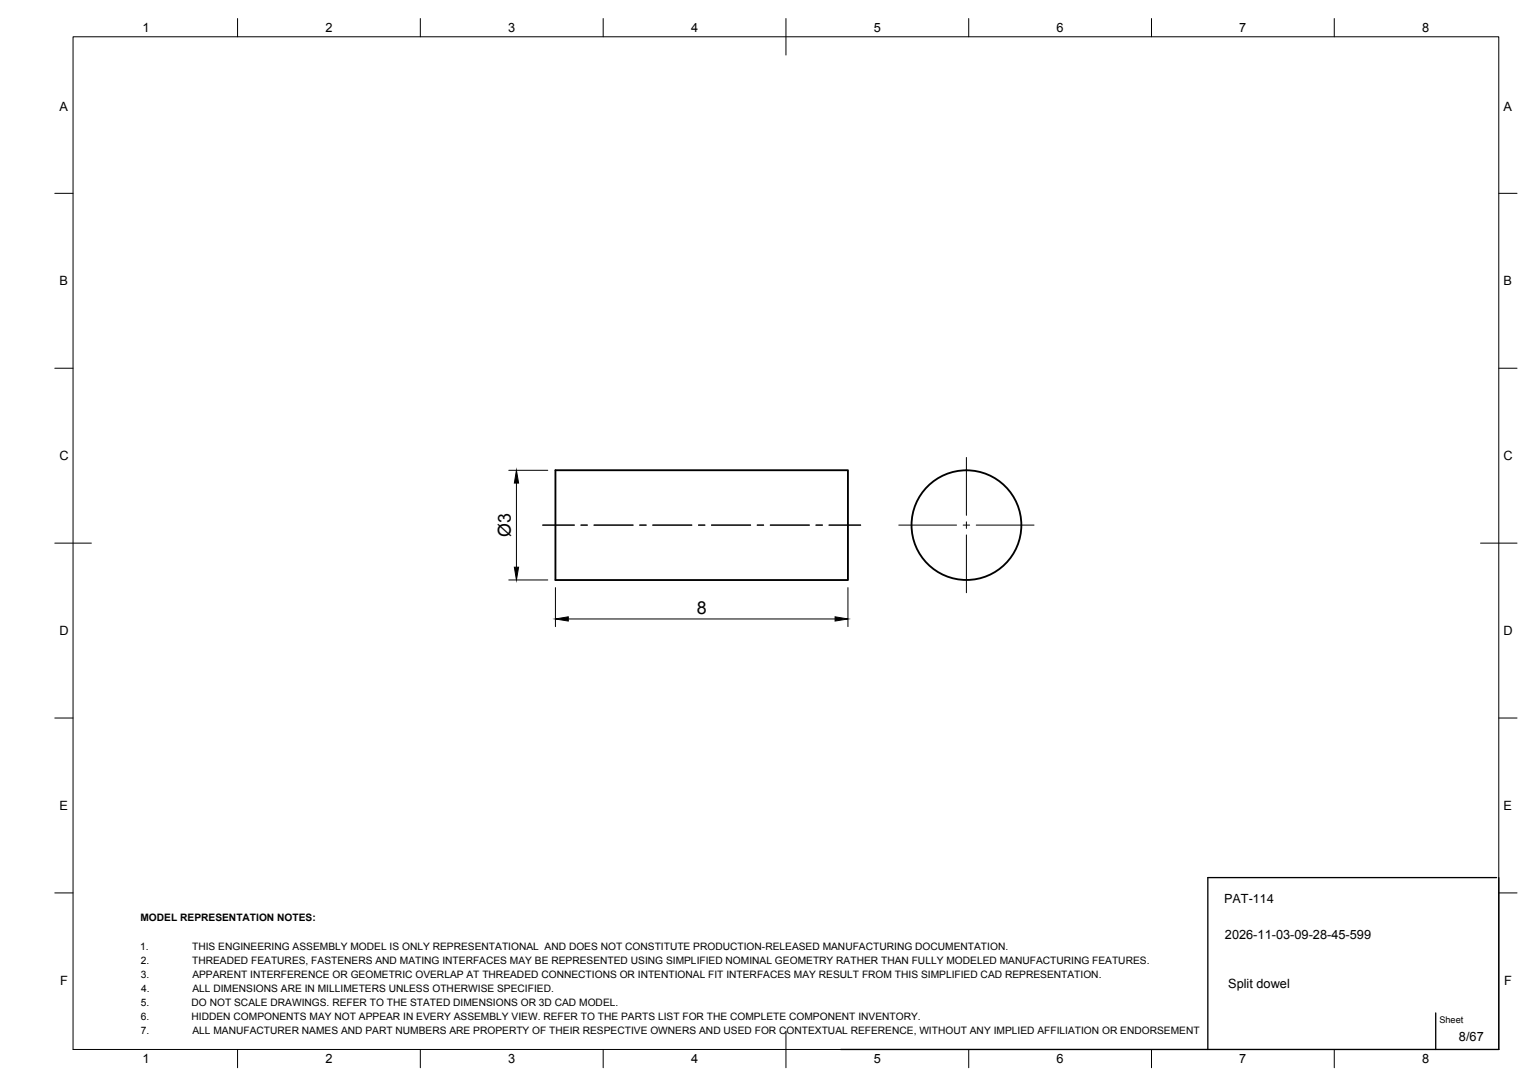
ISO-10303-21;
HEADER;
/* Generated by software containing ST-Developer
 * from STEP Tools, Inc. (www.steptools.com) 
 */

FILE_DESCRIPTION(
/* description */ ('Two-stage gear reducer in split housing'),
/* implementation_level */ '2;1');

FILE_NAME(
/* name */ 'Split dowel.step',
/* time_stamp */ '2026-10-28T03:22:31-07:00',
/* author */ (''),
/* organization */ (''),
/* preprocessor_version */ 'ST-DEVELOPER v20.2',
/* originating_system */ 'Autodesk Translation Framework v15.17.0.0',
/* authorisation */ '');

FILE_SCHEMA (('AUTOMOTIVE_DESIGN { 1 0 10303 214 3 1 1 }'));
ENDSEC;

DATA;
#10=MECHANICAL_DESIGN_GEOMETRIC_PRESENTATION_REPRESENTATION('',(#1237),#73366);
#1125=SHAPE_REPRESENTATION_RELATIONSHIP('SRR','None',#73612,#1181);
#1181=ADVANCED_BREP_SHAPE_REPRESENTATION('',(#1308),#73308);
#1237=STYLED_ITEM('',(#73974),#1308);
#1308=MANIFOLD_SOLID_BREP('Body1',#16125);
#1700=PLANE('',#17171);
#1701=PLANE('',#17172);
#2184=FACE_OUTER_BOUND('',#3183,.T.);
#2185=FACE_OUTER_BOUND('',#3184,.T.);
#2186=FACE_OUTER_BOUND('',#3185,.T.);
#3183=EDGE_LOOP('',(#11347,#11348,#11349,#11350));
#3184=EDGE_LOOP('',(#11351));
#3185=EDGE_LOOP('',(#11352));
#4308=LINE('',#23666,#5332);
#5332=VECTOR('',#19426,0.15);
#6272=CIRCLE('',#17169,0.15);
#6273=CIRCLE('',#17170,0.15);
#7104=VERTEX_POINT('',#23663);
#7105=VERTEX_POINT('',#23665);
#8727=EDGE_CURVE('',#7104,#7104,#6272,.T.);
#8728=EDGE_CURVE('',#7104,#7105,#4308,.T.);
#8729=EDGE_CURVE('',#7105,#7105,#6273,.T.);
#11347=ORIENTED_EDGE('',*,*,#8727,.F.);
#11348=ORIENTED_EDGE('',*,*,#8728,.T.);
#11349=ORIENTED_EDGE('',*,*,#8729,.T.);
#11350=ORIENTED_EDGE('',*,*,#8728,.F.);
#11351=ORIENTED_EDGE('',*,*,#8727,.T.);
#11352=ORIENTED_EDGE('',*,*,#8729,.F.);
#14991=CYLINDRICAL_SURFACE('',#17168,0.15);
#15391=ADVANCED_FACE('',(#2184),#14991,.T.);
#15392=ADVANCED_FACE('',(#2185),#1700,.T.);
#15393=ADVANCED_FACE('',(#2186),#1701,.F.);
#16125=CLOSED_SHELL('',(#15391,#15392,#15393));
#17167=AXIS2_PLACEMENT_3D('',#23661,#19420,#19421);
#17168=AXIS2_PLACEMENT_3D('',#23662,#19422,#19423);
#17169=AXIS2_PLACEMENT_3D('',#23664,#19424,#19425);
#17170=AXIS2_PLACEMENT_3D('',#23667,#19427,#19428);
#17171=AXIS2_PLACEMENT_3D('',#23668,#19429,#19430);
#17172=AXIS2_PLACEMENT_3D('',#23669,#19431,#19432);
#19420=DIRECTION('axis',(0.,0.,1.));
#19421=DIRECTION('refdir',(1.,0.,0.));
#19422=DIRECTION('center_axis',(0.,0.,1.));
#19423=DIRECTION('ref_axis',(1.,0.,0.));
#19424=DIRECTION('center_axis',(0.,0.,1.));
#19425=DIRECTION('ref_axis',(1.,0.,0.));
#19426=DIRECTION('',(0.,0.,-1.));
#19427=DIRECTION('center_axis',(0.,0.,1.));
#19428=DIRECTION('ref_axis',(1.,0.,0.));
#19429=DIRECTION('center_axis',(0.,0.,1.));
#19430=DIRECTION('ref_axis',(1.,0.,0.));
#19431=DIRECTION('center_axis',(0.,0.,1.));
#19432=DIRECTION('ref_axis',(1.,0.,0.));
#23661=CARTESIAN_POINT('',(0.,0.,0.));
#23662=CARTESIAN_POINT('Origin',(-4.75,-3.,9.6));
#23663=CARTESIAN_POINT('',(-4.9,-3.,10.4));
#23664=CARTESIAN_POINT('Origin',(-4.75,-3.,10.4));
#23665=CARTESIAN_POINT('',(-4.9,-3.,9.6));
#23666=CARTESIAN_POINT('',(-4.9,-3.,9.6));
#23667=CARTESIAN_POINT('Origin',(-4.75,-3.,9.6));
#23668=CARTESIAN_POINT('Origin',(-4.75,-3.,10.4));
#23669=CARTESIAN_POINT('Origin',(-4.75,-3.,9.6));
#73244=UNCERTAINTY_MEASURE_WITH_UNIT(LENGTH_MEASURE(0.001),#73367,
'DISTANCE_ACCURACY_VALUE',
'Maximum model space distance between geometric entities at asserted c
onnectivities');
#73302=UNCERTAINTY_MEASURE_WITH_UNIT(LENGTH_MEASURE(0.001),#73367,
'DISTANCE_ACCURACY_VALUE',
'Maximum model space distance between geometric entities at asserted c
onnectivities');
#73308=(
GEOMETRIC_REPRESENTATION_CONTEXT(3)
GLOBAL_UNCERTAINTY_ASSIGNED_CONTEXT((#73244))
GLOBAL_UNIT_ASSIGNED_CONTEXT((#73367,#73369,#73370))
REPRESENTATION_CONTEXT('','3D')
);
#73366=(
GEOMETRIC_REPRESENTATION_CONTEXT(3)
GLOBAL_UNCERTAINTY_ASSIGNED_CONTEXT((#73302))
GLOBAL_UNIT_ASSIGNED_CONTEXT((#73367,#73369,#73370))
REPRESENTATION_CONTEXT('','3D')
);
#73367=(
LENGTH_UNIT()
NAMED_UNIT(*)
SI_UNIT(.CENTI.,.METRE.)
);
#73369=(
NAMED_UNIT(*)
PLANE_ANGLE_UNIT()
SI_UNIT($,.RADIAN.)
);
#73370=(
NAMED_UNIT(*)
SI_UNIT($,.STERADIAN.)
SOLID_ANGLE_UNIT()
);
#73376=SHAPE_DEFINITION_REPRESENTATION(#73439,#73612);
#73439=PRODUCT_DEFINITION_SHAPE('',$,#73676);
#73612=SHAPE_REPRESENTATION('',(#17167),#73308);
#73670=PRODUCT_DEFINITION_CONTEXT('part definition',#73861,'design');
#73676=PRODUCT_DEFINITION('Split dowel','Split dowel',#73739,#73670);
#73739=PRODUCT_DEFINITION_FORMATION('',$,#73868);
#73861=APPLICATION_CONTEXT(
'Core Data for Automotive Mechanical Design Process');
#73862=PRODUCT_CONTEXT('part definition',#73861,'mechanical');
#73868=PRODUCT('Split dowel','Split dowel','Split dowel',(#73862));
#73968=COLOUR_RGB('Light Blue',0.38,0.62,0.78);
#73969=FILL_AREA_STYLE_COLOUR('',#73968);
#73970=FILL_AREA_STYLE('',(#73969));
#73971=SURFACE_STYLE_FILL_AREA(#73970);
#73972=SURFACE_SIDE_STYLE('',(#73971));
#73973=SURFACE_STYLE_USAGE(.BOTH.,#73972);
#73974=PRESENTATION_STYLE_ASSIGNMENT((#73973));
ENDSEC;
END-ISO-10303-21;
